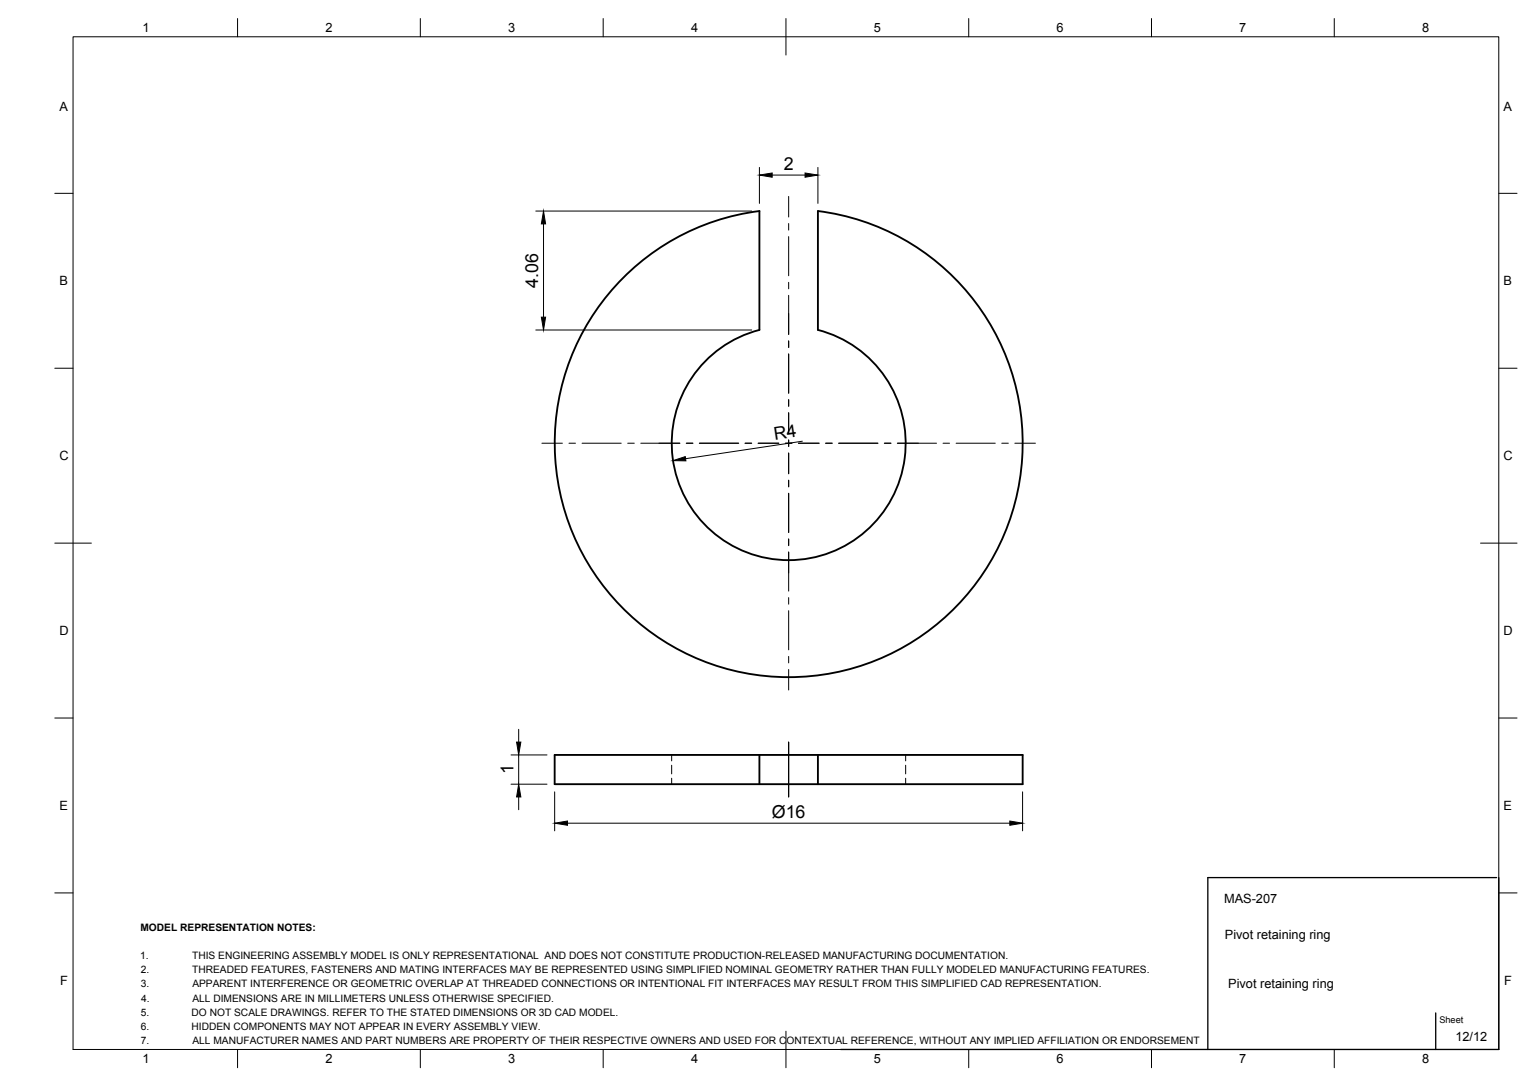
ISO-10303-21;
HEADER;
/* Generated by software containing ST-Developer
 * from STEP Tools, Inc. (www.steptools.com) 
 */

FILE_DESCRIPTION(
/* description */ ('Independent six-slot Geneva indexer. Center distance100, drive radius
50, 60degree indexing per input revolution with120degree engagement an
d240degree dwell. Native machined concave locking faces and relieved d
isk; replaceable retained drive pin; keyed output shaft. Geometry traj
ectory checks use calculated indexing positions, not a contact-dynamic
s simulation. No load or production rating assigned.'),
/* implementation_level */ '2;1');

FILE_NAME(
/* name */ 'Pivot retaining ring.step',
/* time_stamp */ '2026-11-09T17:53:22-08:00',
/* author */ (''),
/* organization */ (''),
/* preprocessor_version */ 'ST-DEVELOPER v20.2',
/* originating_system */ 'Autodesk Translation Framework v15.17.0.0',
/* authorisation */ '');

FILE_SCHEMA (('AUTOMOTIVE_DESIGN { 1 0 10303 214 3 1 1 }'));
ENDSEC;

DATA;
#10=MECHANICAL_DESIGN_GEOMETRIC_PRESENTATION_REPRESENTATION('',(#111),#4149);
#89=SHAPE_REPRESENTATION_RELATIONSHIP('SRR','None',#4206,#100);
#100=ADVANCED_BREP_SHAPE_REPRESENTATION('',(#122),#4148);
#111=STYLED_ITEM('',(#4268),#122);
#122=MANIFOLD_SOLID_BREP('Body1',#2305);
#234=PLANE('',#2690);
#235=PLANE('',#2691);
#236=PLANE('',#2692);
#237=PLANE('',#2699);
#368=FACE_OUTER_BOUND('',#542,.T.);
#369=FACE_OUTER_BOUND('',#543,.T.);
#370=FACE_OUTER_BOUND('',#544,.T.);
#371=FACE_OUTER_BOUND('',#545,.T.);
#372=FACE_OUTER_BOUND('',#546,.T.);
#373=FACE_OUTER_BOUND('',#547,.T.);
#542=EDGE_LOOP('',(#2076,#2077,#2078,#2079));
#543=EDGE_LOOP('',(#2080,#2081,#2082,#2083));
#544=EDGE_LOOP('',(#2084,#2085,#2086,#2087));
#545=EDGE_LOOP('',(#2088,#2089,#2090,#2091));
#546=EDGE_LOOP('',(#2092,#2093,#2094,#2095));
#547=EDGE_LOOP('',(#2096,#2097,#2098,#2099));
#712=LINE('',#4084,#884);
#713=LINE('',#4086,#885);
#714=LINE('',#4088,#886);
#715=LINE('',#4089,#887);
#716=LINE('',#4093,#888);
#717=LINE('',#4095,#889);
#718=LINE('',#4097,#890);
#719=LINE('',#4098,#891);
#884=VECTOR('',#3407,10.);
#885=VECTOR('',#3408,10.);
#886=VECTOR('',#3409,10.);
#887=VECTOR('',#3410,10.);
#888=VECTOR('',#3413,10.);
#889=VECTOR('',#3414,10.);
#890=VECTOR('',#3415,10.);
#891=VECTOR('',#3416,10.);
#1012=CIRCLE('',#2693,8.);
#1013=CIRCLE('',#2694,4.);
#1014=CIRCLE('',#2696,4.);
#1015=CIRCLE('',#2698,8.);
#1204=VERTEX_POINT('',#4082);
#1205=VERTEX_POINT('',#4083);
#1206=VERTEX_POINT('',#4085);
#1207=VERTEX_POINT('',#4087);
#1208=VERTEX_POINT('',#4091);
#1209=VERTEX_POINT('',#4092);
#1210=VERTEX_POINT('',#4094);
#1211=VERTEX_POINT('',#4096);
#1496=EDGE_CURVE('',#1204,#1205,#712,.T.);
#1497=EDGE_CURVE('',#1206,#1204,#713,.T.);
#1498=EDGE_CURVE('',#1207,#1206,#714,.T.);
#1499=EDGE_CURVE('',#1205,#1207,#715,.T.);
#1500=EDGE_CURVE('',#1208,#1209,#716,.T.);
#1501=EDGE_CURVE('',#1210,#1208,#717,.T.);
#1502=EDGE_CURVE('',#1211,#1210,#718,.T.);
#1503=EDGE_CURVE('',#1209,#1211,#719,.T.);
#1504=EDGE_CURVE('',#1206,#1211,#1012,.T.);
#1505=EDGE_CURVE('',#1209,#1204,#1013,.T.);
#1506=EDGE_CURVE('',#1208,#1205,#1014,.T.);
#1507=EDGE_CURVE('',#1207,#1210,#1015,.T.);
#2076=ORIENTED_EDGE('',*,*,#1496,.F.);
#2077=ORIENTED_EDGE('',*,*,#1497,.F.);
#2078=ORIENTED_EDGE('',*,*,#1498,.F.);
#2079=ORIENTED_EDGE('',*,*,#1499,.F.);
#2080=ORIENTED_EDGE('',*,*,#1500,.F.);
#2081=ORIENTED_EDGE('',*,*,#1501,.F.);
#2082=ORIENTED_EDGE('',*,*,#1502,.F.);
#2083=ORIENTED_EDGE('',*,*,#1503,.F.);
#2084=ORIENTED_EDGE('',*,*,#1503,.T.);
#2085=ORIENTED_EDGE('',*,*,#1504,.F.);
#2086=ORIENTED_EDGE('',*,*,#1497,.T.);
#2087=ORIENTED_EDGE('',*,*,#1505,.F.);
#2088=ORIENTED_EDGE('',*,*,#1500,.T.);
#2089=ORIENTED_EDGE('',*,*,#1505,.T.);
#2090=ORIENTED_EDGE('',*,*,#1496,.T.);
#2091=ORIENTED_EDGE('',*,*,#1506,.F.);
#2092=ORIENTED_EDGE('',*,*,#1502,.T.);
#2093=ORIENTED_EDGE('',*,*,#1507,.F.);
#2094=ORIENTED_EDGE('',*,*,#1498,.T.);
#2095=ORIENTED_EDGE('',*,*,#1504,.T.);
#2096=ORIENTED_EDGE('',*,*,#1501,.T.);
#2097=ORIENTED_EDGE('',*,*,#1506,.T.);
#2098=ORIENTED_EDGE('',*,*,#1499,.T.);
#2099=ORIENTED_EDGE('',*,*,#1507,.T.);
#2157=CYLINDRICAL_SURFACE('',#2695,4.);
#2158=CYLINDRICAL_SURFACE('',#2697,8.);
#2289=ADVANCED_FACE('',(#368),#234,.F.);
#2290=ADVANCED_FACE('',(#369),#235,.F.);
#2291=ADVANCED_FACE('',(#370),#236,.F.);
#2292=ADVANCED_FACE('',(#371),#2157,.F.);
#2293=ADVANCED_FACE('',(#372),#2158,.T.);
#2294=ADVANCED_FACE('',(#373),#237,.T.);
#2305=CLOSED_SHELL('',(#2289,#2290,#2291,#2292,#2293,#2294));
#2689=AXIS2_PLACEMENT_3D('',#4080,#3403,#3404);
#2690=AXIS2_PLACEMENT_3D('',#4081,#3405,#3406);
#2691=AXIS2_PLACEMENT_3D('',#4090,#3411,#3412);
#2692=AXIS2_PLACEMENT_3D('',#4099,#3417,#3418);
#2693=AXIS2_PLACEMENT_3D('',#4100,#3419,#3420);
#2694=AXIS2_PLACEMENT_3D('',#4101,#3421,#3422);
#2695=AXIS2_PLACEMENT_3D('',#4102,#3423,#3424);
#2696=AXIS2_PLACEMENT_3D('',#4103,#3425,#3426);
#2697=AXIS2_PLACEMENT_3D('',#4104,#3427,#3428);
#2698=AXIS2_PLACEMENT_3D('',#4105,#3429,#3430);
#2699=AXIS2_PLACEMENT_3D('',#4106,#3431,#3432);
#3403=DIRECTION('axis',(0.,0.,1.));
#3404=DIRECTION('refdir',(1.,0.,0.));
#3405=DIRECTION('center_axis',(-1.,0.,0.));
#3406=DIRECTION('ref_axis',(0.,1.,0.));
#3407=DIRECTION('',(0.,0.,1.));
#3408=DIRECTION('',(0.,-1.,0.));
#3409=DIRECTION('',(0.,0.,-1.));
#3410=DIRECTION('',(0.,1.,0.));
#3411=DIRECTION('center_axis',(1.,0.,0.));
#3412=DIRECTION('ref_axis',(0.,-1.,0.));
#3413=DIRECTION('',(0.,0.,-1.));
#3414=DIRECTION('',(0.,-1.,0.));
#3415=DIRECTION('',(0.,0.,1.));
#3416=DIRECTION('',(0.,1.,0.));
#3417=DIRECTION('center_axis',(0.,0.,1.));
#3418=DIRECTION('ref_axis',(1.,0.,0.));
#3419=DIRECTION('center_axis',(0.,0.,1.));
#3420=DIRECTION('ref_axis',(1.,0.,0.));
#3421=DIRECTION('center_axis',(0.,0.,-1.));
#3422=DIRECTION('ref_axis',(1.,0.,0.));
#3423=DIRECTION('center_axis',(0.,0.,1.));
#3424=DIRECTION('ref_axis',(6.12323399573677E-17,-1.,0.));
#3425=DIRECTION('center_axis',(0.,0.,-1.));
#3426=DIRECTION('ref_axis',(1.,0.,0.));
#3427=DIRECTION('center_axis',(0.,0.,1.));
#3428=DIRECTION('ref_axis',(6.12323399573677E-17,-1.,0.));
#3429=DIRECTION('center_axis',(0.,0.,1.));
#3430=DIRECTION('ref_axis',(1.,0.,0.));
#3431=DIRECTION('center_axis',(0.,0.,1.));
#3432=DIRECTION('ref_axis',(1.,0.,0.));
#4080=CARTESIAN_POINT('',(0.,0.,0.));
#4081=CARTESIAN_POINT('Origin',(-1.,0.,1.));
#4082=CARTESIAN_POINT('',(-1.,3.87298334620742,0.));
#4083=CARTESIAN_POINT('',(-1.,3.87298334620742,1.));
#4084=CARTESIAN_POINT('',(-1.,3.87298334620742,0.));
#4085=CARTESIAN_POINT('',(-1.,7.93725393319377,0.));
#4086=CARTESIAN_POINT('',(-1.,0.,0.));
#4087=CARTESIAN_POINT('',(-1.,7.93725393319377,1.));
#4088=CARTESIAN_POINT('',(-1.,7.93725393319377,0.));
#4089=CARTESIAN_POINT('',(-1.,0.,1.));
#4090=CARTESIAN_POINT('Origin',(1.,16.,1.));
#4091=CARTESIAN_POINT('',(1.,3.87298334620742,1.));
#4092=CARTESIAN_POINT('',(1.,3.87298334620742,0.));
#4093=CARTESIAN_POINT('',(1.,3.87298334620742,0.));
#4094=CARTESIAN_POINT('',(1.,7.93725393319377,1.));
#4095=CARTESIAN_POINT('',(1.,8.,1.));
#4096=CARTESIAN_POINT('',(1.,7.93725393319377,0.));
#4097=CARTESIAN_POINT('',(1.,7.93725393319377,0.));
#4098=CARTESIAN_POINT('',(1.,8.,0.));
#4099=CARTESIAN_POINT('Origin',(0.,0.,0.));
#4100=CARTESIAN_POINT('Origin',(0.,0.,0.));
#4101=CARTESIAN_POINT('Origin',(0.,0.,0.));
#4102=CARTESIAN_POINT('Origin',(0.,0.,0.));
#4103=CARTESIAN_POINT('Origin',(0.,0.,1.));
#4104=CARTESIAN_POINT('Origin',(0.,0.,0.));
#4105=CARTESIAN_POINT('Origin',(0.,0.,1.));
#4106=CARTESIAN_POINT('Origin',(0.,0.,1.));
#4135=UNCERTAINTY_MEASURE_WITH_UNIT(LENGTH_MEASURE(0.01),#4150,
'DISTANCE_ACCURACY_VALUE',
'Maximum model space distance between geometric entities at asserted c
onnectivities');
#4136=UNCERTAINTY_MEASURE_WITH_UNIT(LENGTH_MEASURE(0.01),#4150,
'DISTANCE_ACCURACY_VALUE',
'Maximum model space distance between geometric entities at asserted c
onnectivities');
#4148=(
GEOMETRIC_REPRESENTATION_CONTEXT(3)
GLOBAL_UNCERTAINTY_ASSIGNED_CONTEXT((#4135))
GLOBAL_UNIT_ASSIGNED_CONTEXT((#4150,#4152,#4153))
REPRESENTATION_CONTEXT('','3D')
);
#4149=(
GEOMETRIC_REPRESENTATION_CONTEXT(3)
GLOBAL_UNCERTAINTY_ASSIGNED_CONTEXT((#4136))
GLOBAL_UNIT_ASSIGNED_CONTEXT((#4150,#4152,#4153))
REPRESENTATION_CONTEXT('','3D')
);
#4150=(
LENGTH_UNIT()
NAMED_UNIT(*)
SI_UNIT(.MILLI.,.METRE.)
);
#4152=(
NAMED_UNIT(*)
PLANE_ANGLE_UNIT()
SI_UNIT($,.RADIAN.)
);
#4153=(
NAMED_UNIT(*)
SI_UNIT($,.STERADIAN.)
SOLID_ANGLE_UNIT()
);
#4165=SHAPE_DEFINITION_REPRESENTATION(#4177,#4206);
#4177=PRODUCT_DEFINITION_SHAPE('',$,#4219);
#4206=SHAPE_REPRESENTATION('',(#2689),#4148);
#4207=PRODUCT_DEFINITION_CONTEXT('part definition',#4245,'design');
#4219=PRODUCT_DEFINITION('Pivot retaining ring','Pivot retaining ring',
#4231,#4207);
#4231=PRODUCT_DEFINITION_FORMATION('',$,#4258);
#4245=APPLICATION_CONTEXT(
'Core Data for Automotive Mechanical Design Process');
#4246=PRODUCT_CONTEXT('part definition',#4245,'mechanical');
#4258=PRODUCT('Pivot retaining ring','Pivot retaining ring',$,(#4246));
#4268=PRESENTATION_STYLE_ASSIGNMENT((#4278));
#4278=SURFACE_STYLE_USAGE(.BOTH.,#4288);
#4288=SURFACE_SIDE_STYLE('',(#4298));
#4298=SURFACE_STYLE_FILL_AREA(#4308);
#4308=FILL_AREA_STYLE('Dark gray',(#4318));
#4318=FILL_AREA_STYLE_COLOUR('Dark gray',#4328);
#4328=COLOUR_RGB('Dark gray',0.250980392156863,0.282352941176471,0.32156862745098);
ENDSEC;
END-ISO-10303-21;
